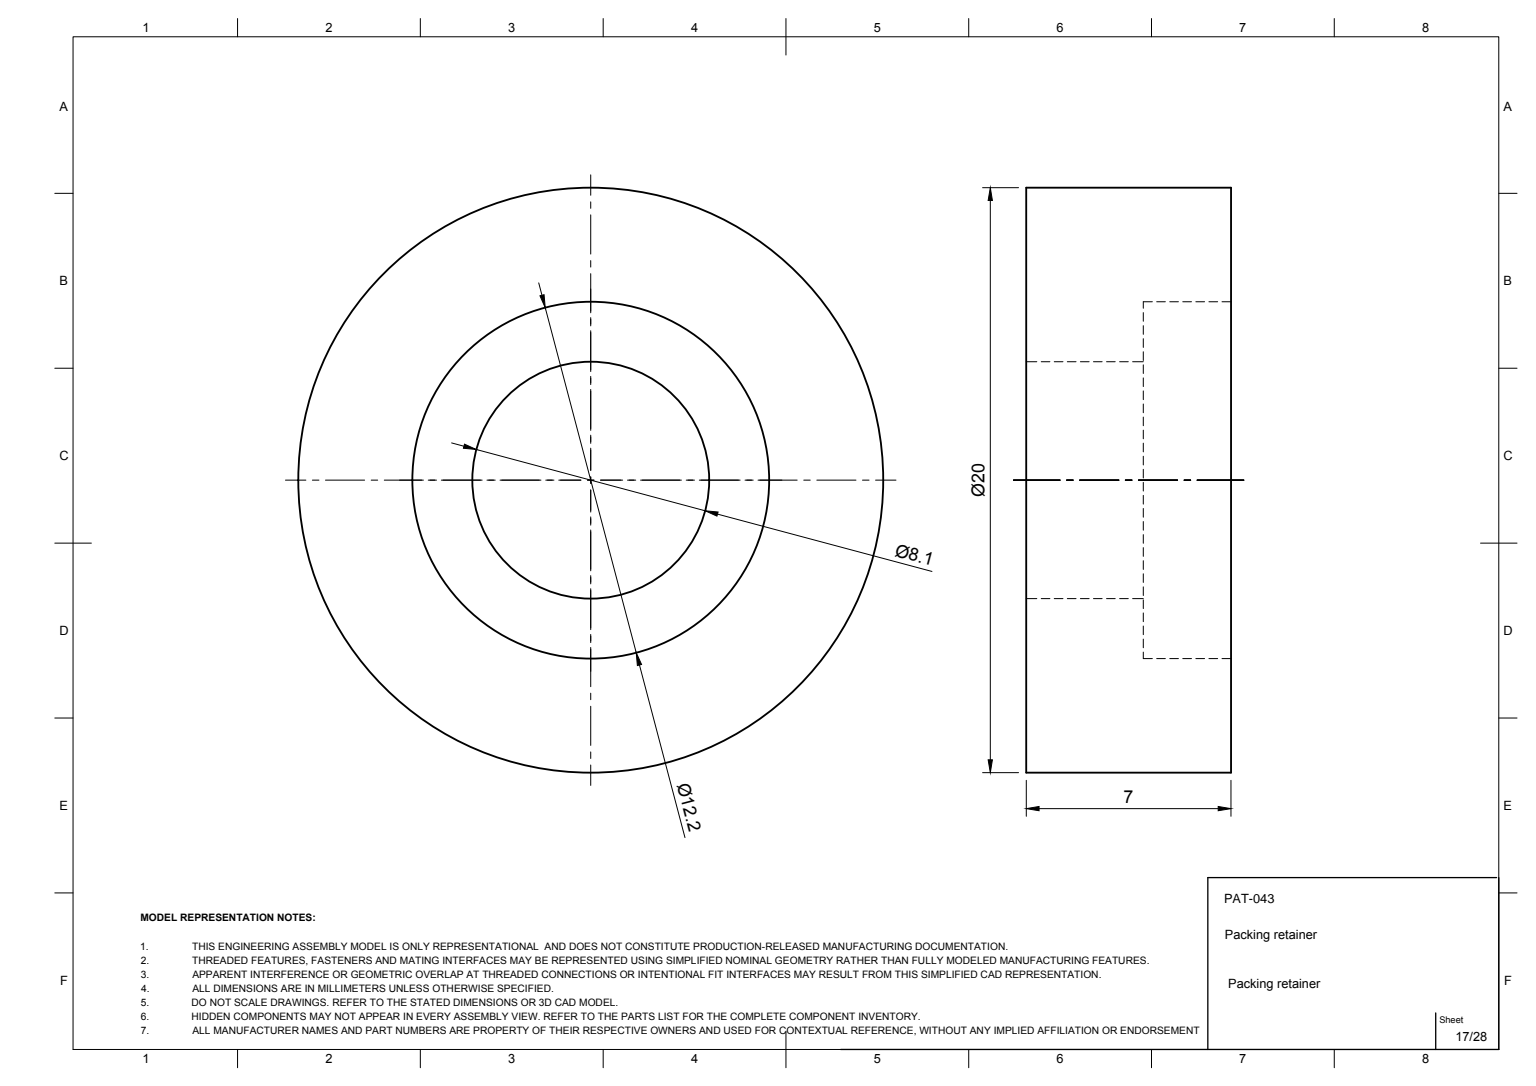
ISO-10303-21;
HEADER;
/* Generated by software containing ST-Developer
 * from STEP Tools, Inc. (www.steptools.com) 
 */

FILE_DESCRIPTION(
/* description */ ('Four-valve pipe header'),
/* implementation_level */ '2;1');

FILE_NAME(
/* name */ 'Packing retainer.step',
/* time_stamp */ '2026-10-29T16:56:19-07:00',
/* author */ (''),
/* organization */ (''),
/* preprocessor_version */ 'ST-DEVELOPER v20.2',
/* originating_system */ 'Autodesk Translation Framework v15.17.0.0',
/* authorisation */ '');

FILE_SCHEMA (('AUTOMOTIVE_DESIGN { 1 0 10303 214 3 1 1 }'));
ENDSEC;

DATA;
#10=MECHANICAL_DESIGN_GEOMETRIC_PRESENTATION_REPRESENTATION('',(#343),#10119);
#291=SHAPE_REPRESENTATION_RELATIONSHIP('SRR','None',#10253,#317);
#317=ADVANCED_BREP_SHAPE_REPRESENTATION('',(#369),#10102);
#343=STYLED_ITEM('',(#10456),#369);
#369=MANIFOLD_SOLID_BREP('Body1',#5589);
#495=FACE_BOUND('',#1318,.T.);
#496=FACE_BOUND('',#1322,.T.);
#497=FACE_BOUND('',#1324,.T.);
#633=PLANE('',#6240);
#634=PLANE('',#6247);
#635=PLANE('',#6248);
#915=FACE_OUTER_BOUND('',#1316,.T.);
#916=FACE_OUTER_BOUND('',#1317,.T.);
#917=FACE_OUTER_BOUND('',#1319,.T.);
#918=FACE_OUTER_BOUND('',#1320,.T.);
#919=FACE_OUTER_BOUND('',#1321,.T.);
#920=FACE_OUTER_BOUND('',#1323,.T.);
#1316=EDGE_LOOP('',(#4505,#4506,#4507,#4508));
#1317=EDGE_LOOP('',(#4509));
#1318=EDGE_LOOP('',(#4510));
#1319=EDGE_LOOP('',(#4511,#4512,#4513,#4514));
#1320=EDGE_LOOP('',(#4515,#4516,#4517,#4518));
#1321=EDGE_LOOP('',(#4519));
#1322=EDGE_LOOP('',(#4520));
#1323=EDGE_LOOP('',(#4521));
#1324=EDGE_LOOP('',(#4522));
#1724=LINE('',#9272,#2142);
#1725=LINE('',#9280,#2143);
#1726=LINE('',#9285,#2144);
#2142=VECTOR('',#7461,0.61);
#2143=VECTOR('',#7472,0.405);
#2144=VECTOR('',#7477,1.);
#2484=CIRCLE('',#6238,0.61);
#2485=CIRCLE('',#6239,0.61);
#2486=CIRCLE('',#6241,0.405);
#2487=CIRCLE('',#6243,0.405);
#2488=CIRCLE('',#6245,1.);
#2489=CIRCLE('',#6246,1.);
#2829=VERTEX_POINT('',#9269);
#2830=VERTEX_POINT('',#9271);
#2831=VERTEX_POINT('',#9275);
#2832=VERTEX_POINT('',#9278);
#2833=VERTEX_POINT('',#9282);
#2834=VERTEX_POINT('',#9284);
#3419=EDGE_CURVE('',#2829,#2829,#2484,.T.);
#3420=EDGE_CURVE('',#2829,#2830,#1724,.T.);
#3421=EDGE_CURVE('',#2830,#2830,#2485,.T.);
#3422=EDGE_CURVE('',#2831,#2831,#2486,.T.);
#3423=EDGE_CURVE('',#2832,#2832,#2487,.T.);
#3424=EDGE_CURVE('',#2832,#2831,#1725,.T.);
#3425=EDGE_CURVE('',#2833,#2833,#2488,.T.);
#3426=EDGE_CURVE('',#2833,#2834,#1726,.T.);
#3427=EDGE_CURVE('',#2834,#2834,#2489,.T.);
#4505=ORIENTED_EDGE('',*,*,#3419,.F.);
#4506=ORIENTED_EDGE('',*,*,#3420,.T.);
#4507=ORIENTED_EDGE('',*,*,#3421,.T.);
#4508=ORIENTED_EDGE('',*,*,#3420,.F.);
#4509=ORIENTED_EDGE('',*,*,#3421,.F.);
#4510=ORIENTED_EDGE('',*,*,#3422,.F.);
#4511=ORIENTED_EDGE('',*,*,#3423,.F.);
#4512=ORIENTED_EDGE('',*,*,#3424,.T.);
#4513=ORIENTED_EDGE('',*,*,#3422,.T.);
#4514=ORIENTED_EDGE('',*,*,#3424,.F.);
#4515=ORIENTED_EDGE('',*,*,#3425,.F.);
#4516=ORIENTED_EDGE('',*,*,#3426,.T.);
#4517=ORIENTED_EDGE('',*,*,#3427,.T.);
#4518=ORIENTED_EDGE('',*,*,#3426,.F.);
#4519=ORIENTED_EDGE('',*,*,#3425,.T.);
#4520=ORIENTED_EDGE('',*,*,#3423,.T.);
#4521=ORIENTED_EDGE('',*,*,#3427,.F.);
#4522=ORIENTED_EDGE('',*,*,#3419,.T.);
#5214=CYLINDRICAL_SURFACE('',#6237,0.61);
#5215=CYLINDRICAL_SURFACE('',#6242,0.405);
#5216=CYLINDRICAL_SURFACE('',#6244,1.);
#5415=ADVANCED_FACE('',(#915),#5214,.F.);
#5416=ADVANCED_FACE('',(#916,#495),#633,.F.);
#5417=ADVANCED_FACE('',(#917),#5215,.F.);
#5418=ADVANCED_FACE('',(#918),#5216,.T.);
#5419=ADVANCED_FACE('',(#919,#496),#634,.T.);
#5420=ADVANCED_FACE('',(#920,#497),#635,.F.);
#5589=CLOSED_SHELL('',(#5415,#5416,#5417,#5418,#5419,#5420));
#6236=AXIS2_PLACEMENT_3D('',#9267,#7455,#7456);
#6237=AXIS2_PLACEMENT_3D('',#9268,#7457,#7458);
#6238=AXIS2_PLACEMENT_3D('',#9270,#7459,#7460);
#6239=AXIS2_PLACEMENT_3D('',#9273,#7462,#7463);
#6240=AXIS2_PLACEMENT_3D('',#9274,#7464,#7465);
#6241=AXIS2_PLACEMENT_3D('',#9276,#7466,#7467);
#6242=AXIS2_PLACEMENT_3D('',#9277,#7468,#7469);
#6243=AXIS2_PLACEMENT_3D('',#9279,#7470,#7471);
#6244=AXIS2_PLACEMENT_3D('',#9281,#7473,#7474);
#6245=AXIS2_PLACEMENT_3D('',#9283,#7475,#7476);
#6246=AXIS2_PLACEMENT_3D('',#9286,#7478,#7479);
#6247=AXIS2_PLACEMENT_3D('',#9287,#7480,#7481);
#6248=AXIS2_PLACEMENT_3D('',#9288,#7482,#7483);
#7455=DIRECTION('axis',(0.,0.,1.));
#7456=DIRECTION('refdir',(1.,0.,0.));
#7457=DIRECTION('center_axis',(0.,0.,1.));
#7458=DIRECTION('ref_axis',(1.,0.,0.));
#7459=DIRECTION('center_axis',(0.,0.,1.));
#7460=DIRECTION('ref_axis',(1.,0.,0.));
#7461=DIRECTION('',(0.,0.,1.));
#7462=DIRECTION('center_axis',(0.,0.,1.));
#7463=DIRECTION('ref_axis',(1.,0.,0.));
#7464=DIRECTION('center_axis',(0.,0.,1.));
#7465=DIRECTION('ref_axis',(1.,0.,0.));
#7466=DIRECTION('center_axis',(0.,0.,-1.));
#7467=DIRECTION('ref_axis',(1.,0.,0.));
#7468=DIRECTION('center_axis',(0.,0.,1.));
#7469=DIRECTION('ref_axis',(1.,0.,0.));
#7470=DIRECTION('center_axis',(0.,0.,-1.));
#7471=DIRECTION('ref_axis',(1.,0.,0.));
#7472=DIRECTION('',(0.,0.,-1.));
#7473=DIRECTION('center_axis',(0.,0.,1.));
#7474=DIRECTION('ref_axis',(1.,0.,0.));
#7475=DIRECTION('center_axis',(0.,0.,1.));
#7476=DIRECTION('ref_axis',(1.,0.,0.));
#7477=DIRECTION('',(0.,0.,-1.));
#7478=DIRECTION('center_axis',(0.,0.,1.));
#7479=DIRECTION('ref_axis',(1.,0.,0.));
#7480=DIRECTION('center_axis',(0.,0.,1.));
#7481=DIRECTION('ref_axis',(1.,0.,0.));
#7482=DIRECTION('center_axis',(0.,0.,1.));
#7483=DIRECTION('ref_axis',(1.,0.,0.));
#9267=CARTESIAN_POINT('',(0.,0.,0.));
#9268=CARTESIAN_POINT('Origin',(0.,0.,7.9));
#9269=CARTESIAN_POINT('',(-0.61,-7.47034547479885E-17,8.));
#9270=CARTESIAN_POINT('Origin',(0.,0.,8.));
#9271=CARTESIAN_POINT('',(-0.61,-7.47034547479885E-17,8.3));
#9272=CARTESIAN_POINT('',(-0.61,-7.47034547479885E-17,7.9));
#9273=CARTESIAN_POINT('Origin',(0.,0.,8.3));
#9274=CARTESIAN_POINT('Origin',(0.,0.,8.3));
#9275=CARTESIAN_POINT('',(-0.405,4.95981953654678E-17,8.3));
#9276=CARTESIAN_POINT('Origin',(0.,0.,8.3));
#9277=CARTESIAN_POINT('Origin',(0.,0.,8.));
#9278=CARTESIAN_POINT('',(-0.405,-4.95981953654678E-17,8.7));
#9279=CARTESIAN_POINT('Origin',(0.,0.,8.7));
#9280=CARTESIAN_POINT('',(-0.405,-4.95981953654678E-17,8.));
#9281=CARTESIAN_POINT('Origin',(0.,0.,8.));
#9282=CARTESIAN_POINT('',(-1.,-1.22464679914735E-16,8.7));
#9283=CARTESIAN_POINT('Origin',(0.,0.,8.7));
#9284=CARTESIAN_POINT('',(-1.,-1.22464679914735E-16,8.));
#9285=CARTESIAN_POINT('',(-1.,-1.22464679914735E-16,8.));
#9286=CARTESIAN_POINT('Origin',(0.,0.,8.));
#9287=CARTESIAN_POINT('Origin',(0.,0.,8.7));
#9288=CARTESIAN_POINT('Origin',(0.,0.,8.));
#10071=UNCERTAINTY_MEASURE_WITH_UNIT(LENGTH_MEASURE(0.001),#10120,
'DISTANCE_ACCURACY_VALUE',
'Maximum model space distance between geometric entities at asserted c
onnectivities');
#10088=UNCERTAINTY_MEASURE_WITH_UNIT(LENGTH_MEASURE(0.001),#10120,
'DISTANCE_ACCURACY_VALUE',
'Maximum model space distance between geometric entities at asserted c
onnectivities');
#10102=(
GEOMETRIC_REPRESENTATION_CONTEXT(3)
GLOBAL_UNCERTAINTY_ASSIGNED_CONTEXT((#10071))
GLOBAL_UNIT_ASSIGNED_CONTEXT((#10120,#10122,#10123))
REPRESENTATION_CONTEXT('','3D')
);
#10119=(
GEOMETRIC_REPRESENTATION_CONTEXT(3)
GLOBAL_UNCERTAINTY_ASSIGNED_CONTEXT((#10088))
GLOBAL_UNIT_ASSIGNED_CONTEXT((#10120,#10122,#10123))
REPRESENTATION_CONTEXT('','3D')
);
#10120=(
LENGTH_UNIT()
NAMED_UNIT(*)
SI_UNIT(.CENTI.,.METRE.)
);
#10122=(
NAMED_UNIT(*)
PLANE_ANGLE_UNIT()
SI_UNIT($,.RADIAN.)
);
#10123=(
NAMED_UNIT(*)
SI_UNIT($,.STERADIAN.)
SOLID_ANGLE_UNIT()
);
#10137=SHAPE_DEFINITION_REPRESENTATION(#10167,#10253);
#10167=PRODUCT_DEFINITION_SHAPE('',$,#10284);
#10253=SHAPE_REPRESENTATION('',(#6236),#10102);
#10270=PRODUCT_DEFINITION_CONTEXT('part definition',#10362,'design');
#10284=PRODUCT_DEFINITION('Packing retainer','Packing retainer',#10314,
#10270);
#10314=PRODUCT_DEFINITION_FORMATION('',$,#10377);
#10362=APPLICATION_CONTEXT(
'Core Data for Automotive Mechanical Design Process');
#10363=PRODUCT_CONTEXT('part definition',#10362,'mechanical');
#10377=PRODUCT('Packing retainer','Packing retainer','Packing retainer',
(#10363));
#10450=COLOUR_RGB('Light Blue',0.38,0.62,0.78);
#10451=FILL_AREA_STYLE_COLOUR('',#10450);
#10452=FILL_AREA_STYLE('',(#10451));
#10453=SURFACE_STYLE_FILL_AREA(#10452);
#10454=SURFACE_SIDE_STYLE('',(#10453));
#10455=SURFACE_STYLE_USAGE(.BOTH.,#10454);
#10456=PRESENTATION_STYLE_ASSIGNMENT((#10455));
ENDSEC;
END-ISO-10303-21;
